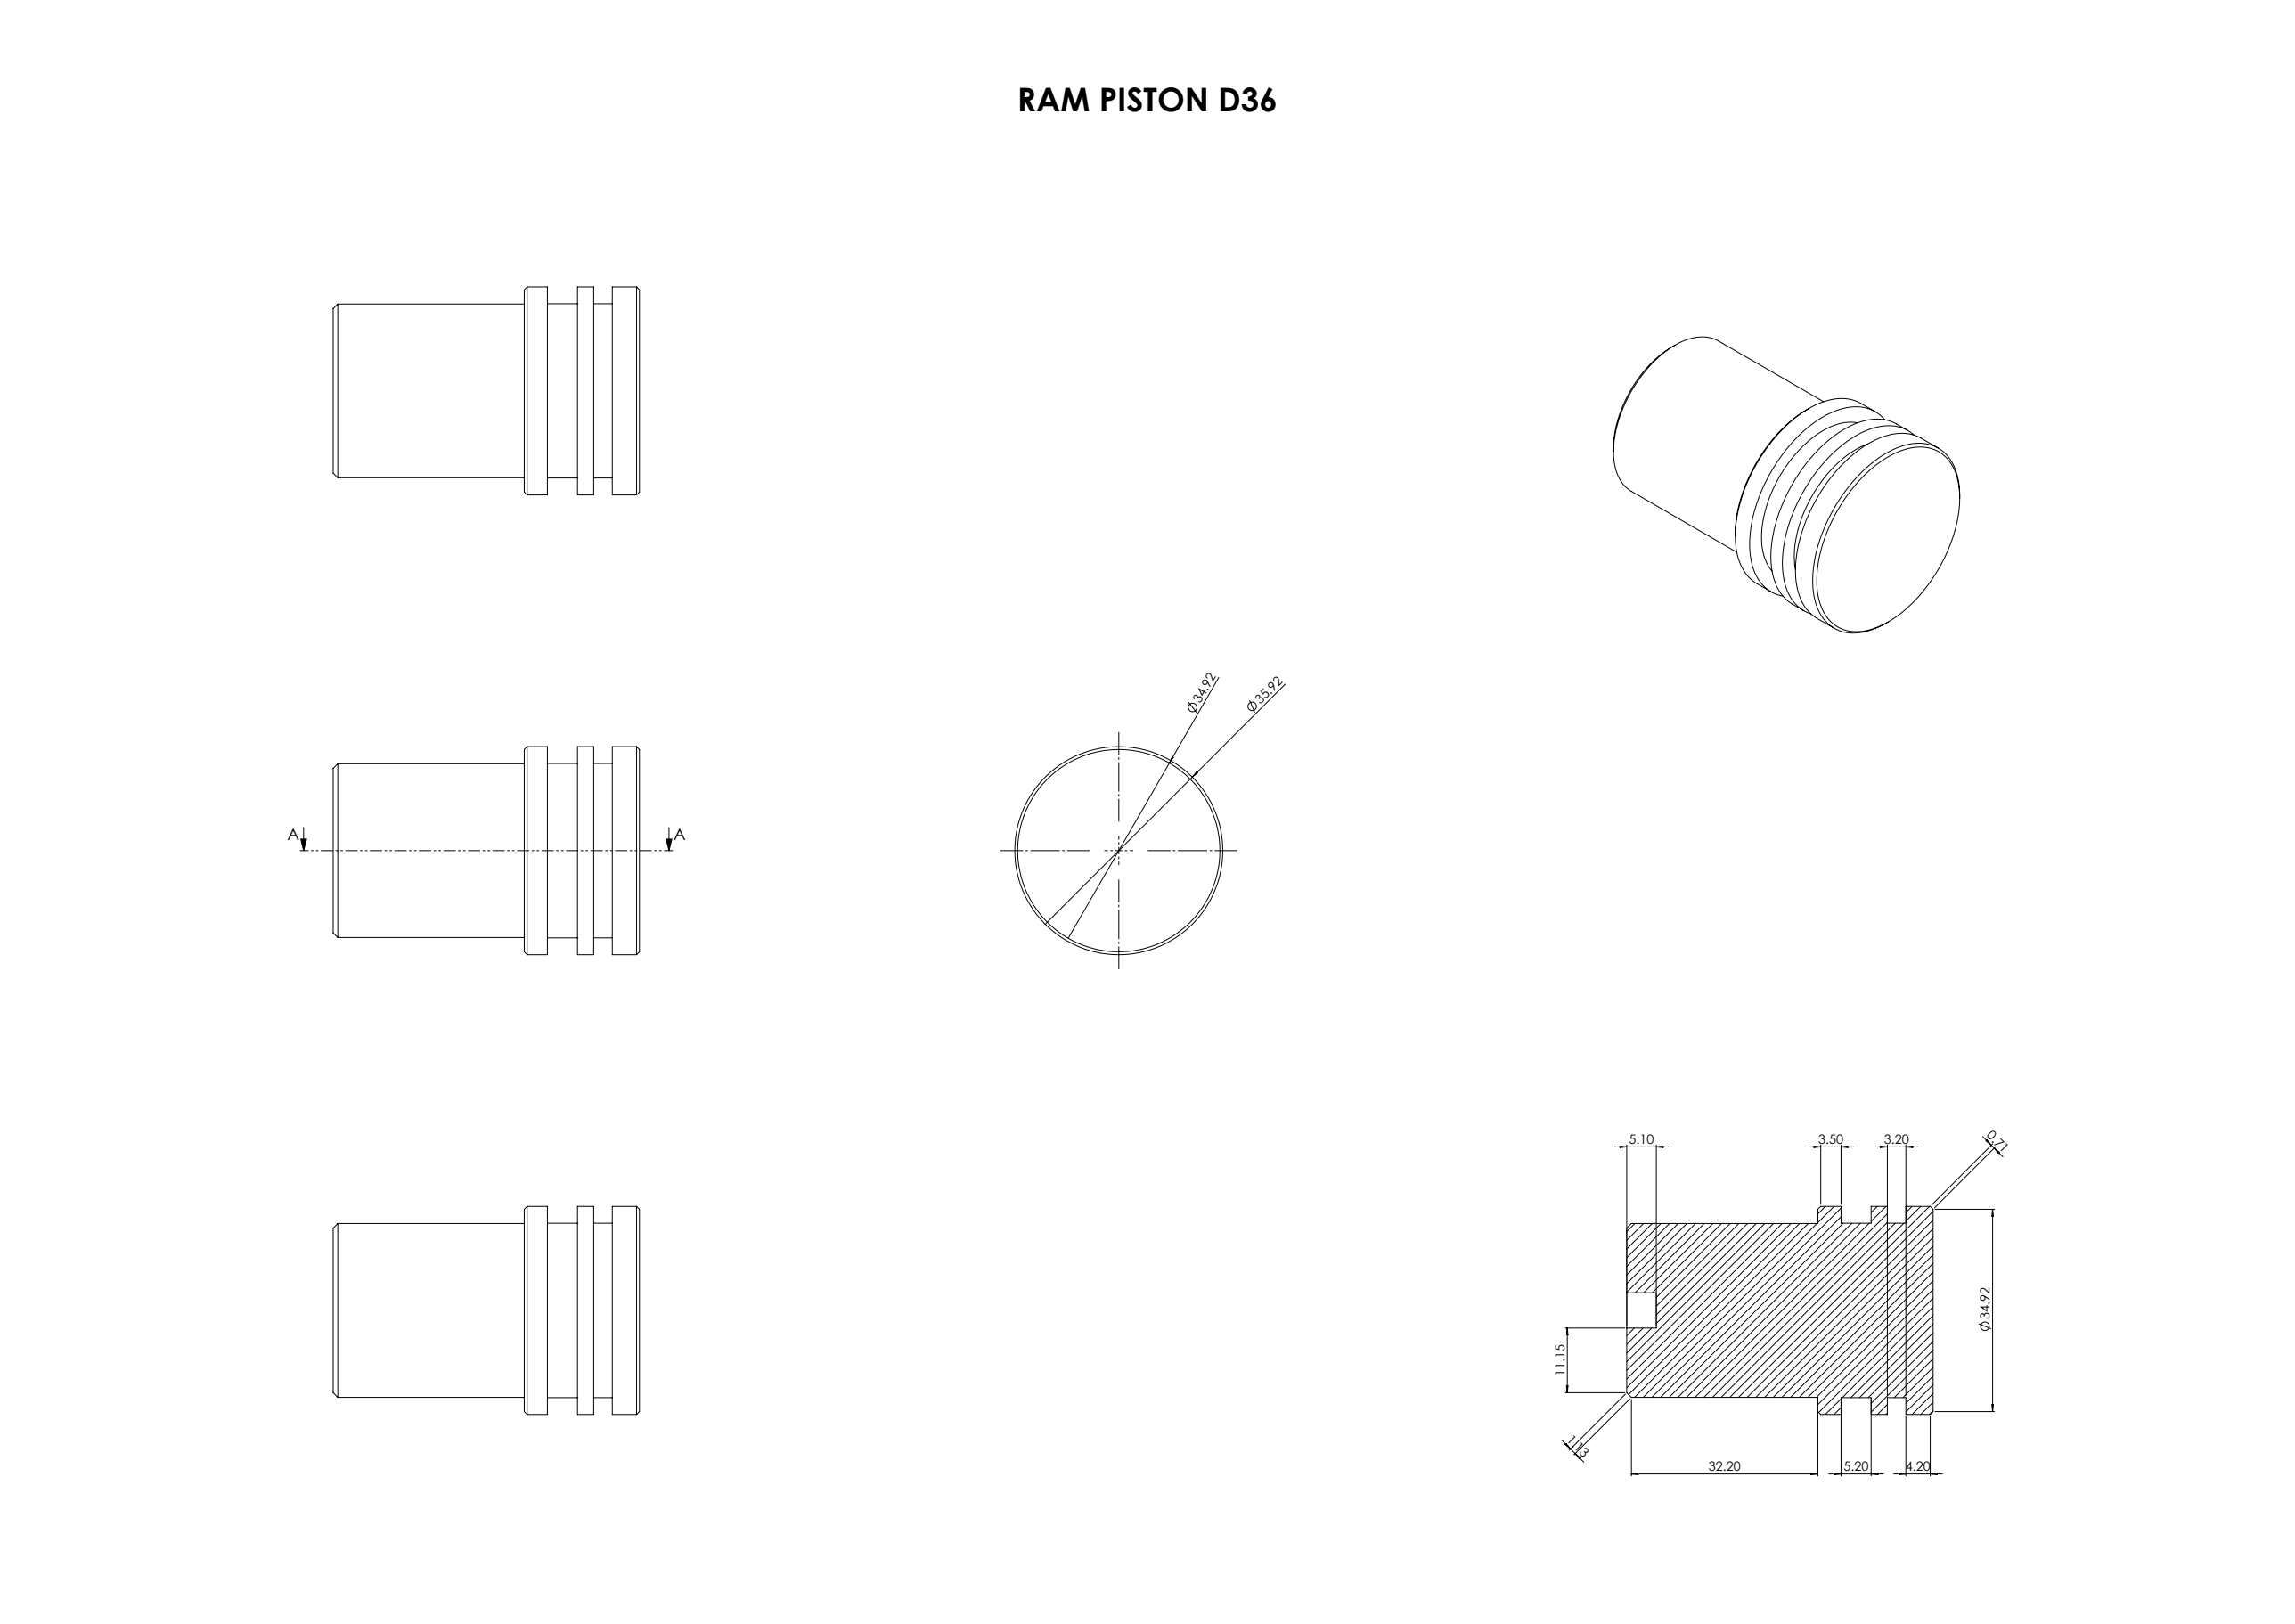
ISO-10303-21;
HEADER;
/* Generated by software containing ST-Developer
 * from STEP Tools, Inc. (www.steptools.com) 
 */

FILE_DESCRIPTION(
/* description */ (''),
/* implementation_level */ '2;1');

FILE_NAME(
/* name */ '03_Ram_Piston_D36.step',
/* time_stamp */ '2026-10-26T03:55:20-07:00',
/* author */ (''),
/* organization */ (''),
/* preprocessor_version */ 'ST-DEVELOPER v20.2',
/* originating_system */ 'Autodesk Translation Framework v15.15.0.0',
/* authorisation */ '');

FILE_SCHEMA (('AUTOMOTIVE_DESIGN { 1 0 10303 214 3 1 1 }'));
ENDSEC;

DATA;
#10=MECHANICAL_DESIGN_GEOMETRIC_PRESENTATION_REPRESENTATION('',(#177),#45236);
#137=SHAPE_REPRESENTATION_RELATIONSHIP('SRR','None',#45316,#157);
#157=ADVANCED_BREP_SHAPE_REPRESENTATION('',(#197),#45218);
#177=STYLED_ITEM('',(#45498),#197);
#197=MANIFOLD_SOLID_BREP('Body1',#16519);
#957=FACE_BOUND('',#3065,.T.);
#958=FACE_BOUND('',#3069,.T.);
#959=FACE_BOUND('',#3073,.T.);
#960=FACE_BOUND('',#3076,.T.);
#961=FACE_BOUND('',#3079,.T.);
#962=FACE_BOUND('',#3082,.T.);
#1122=PLANE('',#17115);
#1123=PLANE('',#17116);
#1124=PLANE('',#17122);
#1125=PLANE('',#17128);
#1126=PLANE('',#17132);
#1127=PLANE('',#17136);
#1128=PLANE('',#17140);
#1129=PLANE('',#17146);
#1674=CYLINDRICAL_SURFACE('',#17112,3.05);
#1675=CYLINDRICAL_SURFACE('',#17120,15.);
#1676=CYLINDRICAL_SURFACE('',#17126,17.96);
#1677=CYLINDRICAL_SURFACE('',#17130,15.05);
#1678=CYLINDRICAL_SURFACE('',#17134,17.96);
#1679=CYLINDRICAL_SURFACE('',#17138,15.05);
#1680=CYLINDRICAL_SURFACE('',#17142,17.96);
#2070=FACE_OUTER_BOUND('',#3062,.T.);
#2071=FACE_OUTER_BOUND('',#3063,.T.);
#2072=FACE_OUTER_BOUND('',#3064,.T.);
#2073=FACE_OUTER_BOUND('',#3066,.T.);
#2074=FACE_OUTER_BOUND('',#3067,.T.);
#2075=FACE_OUTER_BOUND('',#3068,.T.);
#2076=FACE_OUTER_BOUND('',#3070,.T.);
#2077=FACE_OUTER_BOUND('',#3071,.T.);
#2078=FACE_OUTER_BOUND('',#3072,.T.);
#2079=FACE_OUTER_BOUND('',#3074,.T.);
#2080=FACE_OUTER_BOUND('',#3075,.T.);
#2081=FACE_OUTER_BOUND('',#3077,.T.);
#2082=FACE_OUTER_BOUND('',#3078,.T.);
#2083=FACE_OUTER_BOUND('',#3080,.T.);
#2084=FACE_OUTER_BOUND('',#3081,.T.);
#2085=FACE_OUTER_BOUND('',#3083,.T.);
#2086=FACE_OUTER_BOUND('',#3084,.T.);
#2087=FACE_OUTER_BOUND('',#3085,.T.);
#3062=EDGE_LOOP('',(#12074,#12075,#12076,#12077));
#3063=EDGE_LOOP('',(#12078));
#3064=EDGE_LOOP('',(#12079));
#3065=EDGE_LOOP('',(#12080));
#3066=EDGE_LOOP('',(#12081,#12082,#12083,#12084));
#3067=EDGE_LOOP('',(#12085,#12086,#12087,#12088));
#3068=EDGE_LOOP('',(#12089));
#3069=EDGE_LOOP('',(#12090));
#3070=EDGE_LOOP('',(#12091,#12092,#12093,#12094));
#3071=EDGE_LOOP('',(#12095,#12096,#12097,#12098));
#3072=EDGE_LOOP('',(#12099));
#3073=EDGE_LOOP('',(#12100));
#3074=EDGE_LOOP('',(#12101,#12102,#12103,#12104));
#3075=EDGE_LOOP('',(#12105));
#3076=EDGE_LOOP('',(#12106));
#3077=EDGE_LOOP('',(#12107,#12108,#12109,#12110));
#3078=EDGE_LOOP('',(#12111));
#3079=EDGE_LOOP('',(#12112));
#3080=EDGE_LOOP('',(#12113,#12114,#12115,#12116));
#3081=EDGE_LOOP('',(#12117));
#3082=EDGE_LOOP('',(#12118));
#3083=EDGE_LOOP('',(#12119,#12120,#12121,#12122));
#3084=EDGE_LOOP('',(#12123,#12124,#12125,#12126));
#3085=EDGE_LOOP('',(#12127));
#4156=LINE('',#31337,#5467);
#4157=LINE('',#31346,#5468);
#4158=LINE('',#31350,#5469);
#4159=LINE('',#31357,#5470);
#4160=LINE('',#31361,#5471);
#4161=LINE('',#31368,#5472);
#4162=LINE('',#31375,#5473);
#4163=LINE('',#31382,#5474);
#4164=LINE('',#31389,#5475);
#4165=LINE('',#31393,#5476);
#5467=VECTOR('',#19105,3.05);
#5468=VECTOR('',#19118,14.6);
#5469=VECTOR('',#19123,15.);
#5470=VECTOR('',#19132,17.71);
#5471=VECTOR('',#19137,17.96);
#5472=VECTOR('',#19146,15.05);
#5473=VECTOR('',#19155,17.96);
#5474=VECTOR('',#19164,15.05);
#5475=VECTOR('',#19173,17.96);
#5476=VECTOR('',#19178,17.71);
#6644=CIRCLE('',#17113,3.05);
#6645=CIRCLE('',#17114,3.05);
#6646=CIRCLE('',#17117,14.2);
#6647=CIRCLE('',#17119,15.);
#6648=CIRCLE('',#17121,15.);
#6649=CIRCLE('',#17123,17.46);
#6650=CIRCLE('',#17125,17.96);
#6651=CIRCLE('',#17127,17.96);
#6652=CIRCLE('',#17129,15.05);
#6653=CIRCLE('',#17131,15.05);
#6654=CIRCLE('',#17133,17.96);
#6655=CIRCLE('',#17135,17.96);
#6656=CIRCLE('',#17137,15.05);
#6657=CIRCLE('',#17139,15.05);
#6658=CIRCLE('',#17141,17.96);
#6659=CIRCLE('',#17143,17.96);
#6660=CIRCLE('',#17145,17.46);
#7360=VERTEX_POINT('',#31334);
#7361=VERTEX_POINT('',#31336);
#7362=VERTEX_POINT('',#31341);
#7363=VERTEX_POINT('',#31344);
#7364=VERTEX_POINT('',#31348);
#7365=VERTEX_POINT('',#31352);
#7366=VERTEX_POINT('',#31355);
#7367=VERTEX_POINT('',#31359);
#7368=VERTEX_POINT('',#31363);
#7369=VERTEX_POINT('',#31366);
#7370=VERTEX_POINT('',#31370);
#7371=VERTEX_POINT('',#31373);
#7372=VERTEX_POINT('',#31377);
#7373=VERTEX_POINT('',#31380);
#7374=VERTEX_POINT('',#31384);
#7375=VERTEX_POINT('',#31387);
#7376=VERTEX_POINT('',#31391);
#9100=EDGE_CURVE('',#7360,#7360,#6644,.T.);
#9101=EDGE_CURVE('',#7360,#7361,#4156,.T.);
#9102=EDGE_CURVE('',#7361,#7361,#6645,.T.);
#9103=EDGE_CURVE('',#7362,#7362,#6646,.T.);
#9104=EDGE_CURVE('',#7363,#7363,#6647,.T.);
#9105=EDGE_CURVE('',#7363,#7362,#4157,.T.);
#9106=EDGE_CURVE('',#7364,#7364,#6648,.T.);
#9107=EDGE_CURVE('',#7364,#7363,#4158,.T.);
#9108=EDGE_CURVE('',#7365,#7365,#6649,.T.);
#9109=EDGE_CURVE('',#7366,#7366,#6650,.T.);
#9110=EDGE_CURVE('',#7366,#7365,#4159,.T.);
#9111=EDGE_CURVE('',#7367,#7367,#6651,.T.);
#9112=EDGE_CURVE('',#7367,#7366,#4160,.T.);
#9113=EDGE_CURVE('',#7368,#7368,#6652,.T.);
#9114=EDGE_CURVE('',#7369,#7369,#6653,.T.);
#9115=EDGE_CURVE('',#7369,#7368,#4161,.T.);
#9116=EDGE_CURVE('',#7370,#7370,#6654,.T.);
#9117=EDGE_CURVE('',#7371,#7371,#6655,.T.);
#9118=EDGE_CURVE('',#7371,#7370,#4162,.T.);
#9119=EDGE_CURVE('',#7372,#7372,#6656,.T.);
#9120=EDGE_CURVE('',#7373,#7373,#6657,.T.);
#9121=EDGE_CURVE('',#7373,#7372,#4163,.T.);
#9122=EDGE_CURVE('',#7374,#7374,#6658,.T.);
#9123=EDGE_CURVE('',#7375,#7375,#6659,.T.);
#9124=EDGE_CURVE('',#7375,#7374,#4164,.T.);
#9125=EDGE_CURVE('',#7376,#7376,#6660,.T.);
#9126=EDGE_CURVE('',#7376,#7375,#4165,.T.);
#12074=ORIENTED_EDGE('',*,*,#9100,.F.);
#12075=ORIENTED_EDGE('',*,*,#9101,.T.);
#12076=ORIENTED_EDGE('',*,*,#9102,.T.);
#12077=ORIENTED_EDGE('',*,*,#9101,.F.);
#12078=ORIENTED_EDGE('',*,*,#9102,.F.);
#12079=ORIENTED_EDGE('',*,*,#9103,.F.);
#12080=ORIENTED_EDGE('',*,*,#9100,.T.);
#12081=ORIENTED_EDGE('',*,*,#9104,.F.);
#12082=ORIENTED_EDGE('',*,*,#9105,.T.);
#12083=ORIENTED_EDGE('',*,*,#9103,.T.);
#12084=ORIENTED_EDGE('',*,*,#9105,.F.);
#12085=ORIENTED_EDGE('',*,*,#9106,.F.);
#12086=ORIENTED_EDGE('',*,*,#9107,.T.);
#12087=ORIENTED_EDGE('',*,*,#9104,.T.);
#12088=ORIENTED_EDGE('',*,*,#9107,.F.);
#12089=ORIENTED_EDGE('',*,*,#9108,.F.);
#12090=ORIENTED_EDGE('',*,*,#9106,.T.);
#12091=ORIENTED_EDGE('',*,*,#9109,.F.);
#12092=ORIENTED_EDGE('',*,*,#9110,.T.);
#12093=ORIENTED_EDGE('',*,*,#9108,.T.);
#12094=ORIENTED_EDGE('',*,*,#9110,.F.);
#12095=ORIENTED_EDGE('',*,*,#9111,.F.);
#12096=ORIENTED_EDGE('',*,*,#9112,.T.);
#12097=ORIENTED_EDGE('',*,*,#9109,.T.);
#12098=ORIENTED_EDGE('',*,*,#9112,.F.);
#12099=ORIENTED_EDGE('',*,*,#9111,.T.);
#12100=ORIENTED_EDGE('',*,*,#9113,.F.);
#12101=ORIENTED_EDGE('',*,*,#9114,.F.);
#12102=ORIENTED_EDGE('',*,*,#9115,.T.);
#12103=ORIENTED_EDGE('',*,*,#9113,.T.);
#12104=ORIENTED_EDGE('',*,*,#9115,.F.);
#12105=ORIENTED_EDGE('',*,*,#9116,.F.);
#12106=ORIENTED_EDGE('',*,*,#9114,.T.);
#12107=ORIENTED_EDGE('',*,*,#9117,.F.);
#12108=ORIENTED_EDGE('',*,*,#9118,.T.);
#12109=ORIENTED_EDGE('',*,*,#9116,.T.);
#12110=ORIENTED_EDGE('',*,*,#9118,.F.);
#12111=ORIENTED_EDGE('',*,*,#9117,.T.);
#12112=ORIENTED_EDGE('',*,*,#9119,.F.);
#12113=ORIENTED_EDGE('',*,*,#9120,.F.);
#12114=ORIENTED_EDGE('',*,*,#9121,.T.);
#12115=ORIENTED_EDGE('',*,*,#9119,.T.);
#12116=ORIENTED_EDGE('',*,*,#9121,.F.);
#12117=ORIENTED_EDGE('',*,*,#9122,.F.);
#12118=ORIENTED_EDGE('',*,*,#9120,.T.);
#12119=ORIENTED_EDGE('',*,*,#9123,.F.);
#12120=ORIENTED_EDGE('',*,*,#9124,.T.);
#12121=ORIENTED_EDGE('',*,*,#9122,.T.);
#12122=ORIENTED_EDGE('',*,*,#9124,.F.);
#12123=ORIENTED_EDGE('',*,*,#9125,.F.);
#12124=ORIENTED_EDGE('',*,*,#9126,.T.);
#12125=ORIENTED_EDGE('',*,*,#9123,.T.);
#12126=ORIENTED_EDGE('',*,*,#9126,.F.);
#12127=ORIENTED_EDGE('',*,*,#9125,.T.);
#15495=CONICAL_SURFACE('',#17118,14.6,0.785398163397454);
#15496=CONICAL_SURFACE('',#17124,17.71,0.785398163397442);
#15497=CONICAL_SURFACE('',#17144,17.71,0.785398163397459);
#15798=ADVANCED_FACE('',(#2070),#1674,.F.);
#15799=ADVANCED_FACE('',(#2071),#1122,.F.);
#15800=ADVANCED_FACE('',(#2072,#957),#1123,.T.);
#15801=ADVANCED_FACE('',(#2073),#15495,.T.);
#15802=ADVANCED_FACE('',(#2074),#1675,.T.);
#15803=ADVANCED_FACE('',(#2075,#958),#1124,.T.);
#15804=ADVANCED_FACE('',(#2076),#15496,.T.);
#15805=ADVANCED_FACE('',(#2077),#1676,.T.);
#15806=ADVANCED_FACE('',(#2078,#959),#1125,.T.);
#15807=ADVANCED_FACE('',(#2079),#1677,.T.);
#15808=ADVANCED_FACE('',(#2080,#960),#1126,.T.);
#15809=ADVANCED_FACE('',(#2081),#1678,.T.);
#15810=ADVANCED_FACE('',(#2082,#961),#1127,.T.);
#15811=ADVANCED_FACE('',(#2083),#1679,.T.);
#15812=ADVANCED_FACE('',(#2084,#962),#1128,.T.);
#15813=ADVANCED_FACE('',(#2085),#1680,.T.);
#15814=ADVANCED_FACE('',(#2086),#15497,.T.);
#15815=ADVANCED_FACE('',(#2087),#1129,.T.);
#16519=CLOSED_SHELL('',(#15798,#15799,#15800,#15801,#15802,#15803,#15804,
#15805,#15806,#15807,#15808,#15809,#15810,#15811,#15812,#15813,#15814,#15815));
#17111=AXIS2_PLACEMENT_3D('',#31332,#19099,#19100);
#17112=AXIS2_PLACEMENT_3D('',#31333,#19101,#19102);
#17113=AXIS2_PLACEMENT_3D('',#31335,#19103,#19104);
#17114=AXIS2_PLACEMENT_3D('',#31338,#19106,#19107);
#17115=AXIS2_PLACEMENT_3D('',#31339,#19108,#19109);
#17116=AXIS2_PLACEMENT_3D('',#31340,#19110,#19111);
#17117=AXIS2_PLACEMENT_3D('',#31342,#19112,#19113);
#17118=AXIS2_PLACEMENT_3D('',#31343,#19114,#19115);
#17119=AXIS2_PLACEMENT_3D('',#31345,#19116,#19117);
#17120=AXIS2_PLACEMENT_3D('',#31347,#19119,#19120);
#17121=AXIS2_PLACEMENT_3D('',#31349,#19121,#19122);
#17122=AXIS2_PLACEMENT_3D('',#31351,#19124,#19125);
#17123=AXIS2_PLACEMENT_3D('',#31353,#19126,#19127);
#17124=AXIS2_PLACEMENT_3D('',#31354,#19128,#19129);
#17125=AXIS2_PLACEMENT_3D('',#31356,#19130,#19131);
#17126=AXIS2_PLACEMENT_3D('',#31358,#19133,#19134);
#17127=AXIS2_PLACEMENT_3D('',#31360,#19135,#19136);
#17128=AXIS2_PLACEMENT_3D('',#31362,#19138,#19139);
#17129=AXIS2_PLACEMENT_3D('',#31364,#19140,#19141);
#17130=AXIS2_PLACEMENT_3D('',#31365,#19142,#19143);
#17131=AXIS2_PLACEMENT_3D('',#31367,#19144,#19145);
#17132=AXIS2_PLACEMENT_3D('',#31369,#19147,#19148);
#17133=AXIS2_PLACEMENT_3D('',#31371,#19149,#19150);
#17134=AXIS2_PLACEMENT_3D('',#31372,#19151,#19152);
#17135=AXIS2_PLACEMENT_3D('',#31374,#19153,#19154);
#17136=AXIS2_PLACEMENT_3D('',#31376,#19156,#19157);
#17137=AXIS2_PLACEMENT_3D('',#31378,#19158,#19159);
#17138=AXIS2_PLACEMENT_3D('',#31379,#19160,#19161);
#17139=AXIS2_PLACEMENT_3D('',#31381,#19162,#19163);
#17140=AXIS2_PLACEMENT_3D('',#31383,#19165,#19166);
#17141=AXIS2_PLACEMENT_3D('',#31385,#19167,#19168);
#17142=AXIS2_PLACEMENT_3D('',#31386,#19169,#19170);
#17143=AXIS2_PLACEMENT_3D('',#31388,#19171,#19172);
#17144=AXIS2_PLACEMENT_3D('',#31390,#19174,#19175);
#17145=AXIS2_PLACEMENT_3D('',#31392,#19176,#19177);
#17146=AXIS2_PLACEMENT_3D('',#31394,#19179,#19180);
#19099=DIRECTION('axis',(0.,0.,1.));
#19100=DIRECTION('refdir',(1.,0.,0.));
#19101=DIRECTION('center_axis',(1.,0.,0.));
#19102=DIRECTION('ref_axis',(0.,0.,-1.));
#19103=DIRECTION('center_axis',(1.,0.,0.));
#19104=DIRECTION('ref_axis',(0.,0.,-1.));
#19105=DIRECTION('',(1.,0.,0.));
#19106=DIRECTION('center_axis',(1.,0.,0.));
#19107=DIRECTION('ref_axis',(0.,0.,-1.));
#19108=DIRECTION('center_axis',(1.,0.,0.));
#19109=DIRECTION('ref_axis',(0.,0.,-1.));
#19110=DIRECTION('center_axis',(-1.,0.,0.));
#19111=DIRECTION('ref_axis',(0.,0.,1.));
#19112=DIRECTION('center_axis',(1.,0.,0.));
#19113=DIRECTION('ref_axis',(0.,0.,-1.));
#19114=DIRECTION('center_axis',(1.,0.,0.));
#19115=DIRECTION('ref_axis',(0.,1.,0.));
#19116=DIRECTION('center_axis',(1.,0.,0.));
#19117=DIRECTION('ref_axis',(0.,0.,-1.));
#19118=DIRECTION('',(-0.707106781186544,0.707106781186551,8.65956056235498E-17));
#19119=DIRECTION('center_axis',(1.,0.,0.));
#19120=DIRECTION('ref_axis',(0.,1.,0.));
#19121=DIRECTION('center_axis',(1.,0.,0.));
#19122=DIRECTION('ref_axis',(0.,0.,-1.));
#19123=DIRECTION('',(-1.,0.,0.));
#19124=DIRECTION('center_axis',(-1.,0.,0.));
#19125=DIRECTION('ref_axis',(0.,0.,1.));
#19126=DIRECTION('center_axis',(1.,0.,0.));
#19127=DIRECTION('ref_axis',(0.,0.,-1.));
#19128=DIRECTION('center_axis',(1.,0.,0.));
#19129=DIRECTION('ref_axis',(0.,1.,0.));
#19130=DIRECTION('center_axis',(1.,0.,0.));
#19131=DIRECTION('ref_axis',(0.,0.,-1.));
#19132=DIRECTION('',(-0.707106781186552,0.707106781186543,8.65956056235487E-17));
#19133=DIRECTION('center_axis',(1.,0.,0.));
#19134=DIRECTION('ref_axis',(0.,1.,0.));
#19135=DIRECTION('center_axis',(1.,0.,0.));
#19136=DIRECTION('ref_axis',(0.,0.,-1.));
#19137=DIRECTION('',(-1.,0.,0.));
#19138=DIRECTION('center_axis',(1.,0.,0.));
#19139=DIRECTION('ref_axis',(0.,0.,-1.));
#19140=DIRECTION('center_axis',(1.,0.,0.));
#19141=DIRECTION('ref_axis',(0.,0.,-1.));
#19142=DIRECTION('center_axis',(1.,0.,0.));
#19143=DIRECTION('ref_axis',(0.,1.,0.));
#19144=DIRECTION('center_axis',(1.,0.,0.));
#19145=DIRECTION('ref_axis',(0.,0.,-1.));
#19146=DIRECTION('',(-1.,0.,0.));
#19147=DIRECTION('center_axis',(-1.,0.,0.));
#19148=DIRECTION('ref_axis',(0.,0.,1.));
#19149=DIRECTION('center_axis',(1.,0.,0.));
#19150=DIRECTION('ref_axis',(0.,0.,-1.));
#19151=DIRECTION('center_axis',(1.,0.,0.));
#19152=DIRECTION('ref_axis',(0.,1.,0.));
#19153=DIRECTION('center_axis',(1.,0.,0.));
#19154=DIRECTION('ref_axis',(0.,0.,-1.));
#19155=DIRECTION('',(-1.,0.,0.));
#19156=DIRECTION('center_axis',(1.,0.,0.));
#19157=DIRECTION('ref_axis',(0.,0.,-1.));
#19158=DIRECTION('center_axis',(1.,0.,0.));
#19159=DIRECTION('ref_axis',(0.,0.,-1.));
#19160=DIRECTION('center_axis',(1.,0.,0.));
#19161=DIRECTION('ref_axis',(0.,1.,0.));
#19162=DIRECTION('center_axis',(1.,0.,0.));
#19163=DIRECTION('ref_axis',(0.,0.,-1.));
#19164=DIRECTION('',(-1.,0.,0.));
#19165=DIRECTION('center_axis',(-1.,0.,0.));
#19166=DIRECTION('ref_axis',(0.,0.,1.));
#19167=DIRECTION('center_axis',(1.,0.,0.));
#19168=DIRECTION('ref_axis',(0.,0.,-1.));
#19169=DIRECTION('center_axis',(1.,0.,0.));
#19170=DIRECTION('ref_axis',(0.,1.,0.));
#19171=DIRECTION('center_axis',(1.,0.,0.));
#19172=DIRECTION('ref_axis',(0.,0.,-1.));
#19173=DIRECTION('',(-1.,0.,0.));
#19174=DIRECTION('center_axis',(-1.,0.,0.));
#19175=DIRECTION('ref_axis',(0.,1.,0.));
#19176=DIRECTION('center_axis',(1.,0.,0.));
#19177=DIRECTION('ref_axis',(0.,0.,-1.));
#19178=DIRECTION('',(-0.70710678118654,-0.707106781186555,-8.65956056235503E-17));
#19179=DIRECTION('center_axis',(1.,0.,0.));
#19180=DIRECTION('ref_axis',(0.,0.,-1.));
#31332=CARTESIAN_POINT('',(0.,0.,0.));
#31333=CARTESIAN_POINT('Origin',(57.,0.,0.));
#31334=CARTESIAN_POINT('',(57.,-3.73517273739943E-16,3.05));
#31335=CARTESIAN_POINT('Origin',(57.,0.,0.));
#31336=CARTESIAN_POINT('',(62.1,-3.73517273739943E-16,3.05));
#31337=CARTESIAN_POINT('',(57.,-3.73517273739943E-16,3.05));
#31338=CARTESIAN_POINT('Origin',(62.1,0.,0.));
#31339=CARTESIAN_POINT('Origin',(62.1,0.,0.));
#31340=CARTESIAN_POINT('Origin',(57.,14.2,0.));
#31341=CARTESIAN_POINT('',(57.,-14.2,-1.73899845478924E-15));
#31342=CARTESIAN_POINT('Origin',(57.,0.,0.));
#31343=CARTESIAN_POINT('Origin',(57.4,0.,0.));
#31344=CARTESIAN_POINT('',(57.8,-15.,-1.83697019872103E-15));
#31345=CARTESIAN_POINT('Origin',(57.8,0.,0.));
#31346=CARTESIAN_POINT('',(57.4,-14.6,-1.78798432675514E-15));
#31347=CARTESIAN_POINT('Origin',(73.9,0.,0.));
#31348=CARTESIAN_POINT('',(90.,-15.,-1.83697019872103E-15));
#31349=CARTESIAN_POINT('Origin',(90.,0.,0.));
#31350=CARTESIAN_POINT('',(73.9,-15.,-1.83697019872103E-15));
#31351=CARTESIAN_POINT('Origin',(90.,17.46,0.));
#31352=CARTESIAN_POINT('',(90.,-17.46,-2.13823331131128E-15));
#31353=CARTESIAN_POINT('Origin',(90.,0.,0.));
#31354=CARTESIAN_POINT('Origin',(90.25,0.,0.));
#31355=CARTESIAN_POINT('',(90.5,-17.96,-2.19946565126865E-15));
#31356=CARTESIAN_POINT('Origin',(90.5,0.,0.));
#31357=CARTESIAN_POINT('',(90.25,-17.71,-2.16884948128996E-15));
#31358=CARTESIAN_POINT('Origin',(92.25,0.,0.));
#31359=CARTESIAN_POINT('',(94.,-17.96,-2.19946565126865E-15));
#31360=CARTESIAN_POINT('Origin',(94.,0.,0.));
#31361=CARTESIAN_POINT('',(92.25,-17.96,-2.19946565126865E-15));
#31362=CARTESIAN_POINT('Origin',(94.,15.05,0.));
#31363=CARTESIAN_POINT('',(94.,-15.05,-1.84309343271677E-15));
#31364=CARTESIAN_POINT('Origin',(94.,0.,0.));
#31365=CARTESIAN_POINT('Origin',(96.6,0.,0.));
#31366=CARTESIAN_POINT('',(99.2,-15.05,-1.84309343271677E-15));
#31367=CARTESIAN_POINT('Origin',(99.2,0.,0.));
#31368=CARTESIAN_POINT('',(96.6,-15.05,-1.84309343271677E-15));
#31369=CARTESIAN_POINT('Origin',(99.2,17.96,0.));
#31370=CARTESIAN_POINT('',(99.2,-17.96,-2.19946565126865E-15));
#31371=CARTESIAN_POINT('Origin',(99.2,0.,0.));
#31372=CARTESIAN_POINT('Origin',(100.6,0.,0.));
#31373=CARTESIAN_POINT('',(102.,-17.96,-2.19946565126865E-15));
#31374=CARTESIAN_POINT('Origin',(102.,0.,0.));
#31375=CARTESIAN_POINT('',(100.6,-17.96,-2.19946565126865E-15));
#31376=CARTESIAN_POINT('Origin',(102.,15.05,0.));
#31377=CARTESIAN_POINT('',(102.,-15.05,-1.84309343271677E-15));
#31378=CARTESIAN_POINT('Origin',(102.,0.,0.));
#31379=CARTESIAN_POINT('Origin',(103.6,0.,0.));
#31380=CARTESIAN_POINT('',(105.2,-15.05,-1.84309343271677E-15));
#31381=CARTESIAN_POINT('Origin',(105.2,0.,0.));
#31382=CARTESIAN_POINT('',(103.6,-15.05,-1.84309343271677E-15));
#31383=CARTESIAN_POINT('Origin',(105.2,17.96,0.));
#31384=CARTESIAN_POINT('',(105.2,-17.96,-2.19946565126865E-15));
#31385=CARTESIAN_POINT('Origin',(105.2,0.,0.));
#31386=CARTESIAN_POINT('Origin',(107.3,0.,0.));
#31387=CARTESIAN_POINT('',(109.4,-17.96,-2.19946565126865E-15));
#31388=CARTESIAN_POINT('Origin',(109.4,0.,0.));
#31389=CARTESIAN_POINT('',(107.3,-17.96,-2.19946565126865E-15));
#31390=CARTESIAN_POINT('Origin',(109.65,0.,0.));
#31391=CARTESIAN_POINT('',(109.9,-17.46,-2.13823331131128E-15));
#31392=CARTESIAN_POINT('Origin',(109.9,0.,0.));
#31393=CARTESIAN_POINT('',(109.65,-17.71,-2.16884948128996E-15));
#31394=CARTESIAN_POINT('Origin',(109.9,0.,0.));
#45196=UNCERTAINTY_MEASURE_WITH_UNIT(LENGTH_MEASURE(0.01),#45237,
'DISTANCE_ACCURACY_VALUE',
'Maximum model space distance between geometric entities at asserted c
onnectivities');
#45214=UNCERTAINTY_MEASURE_WITH_UNIT(LENGTH_MEASURE(0.01),#45237,
'DISTANCE_ACCURACY_VALUE',
'Maximum model space distance between geometric entities at asserted c
onnectivities');
#45218=(
GEOMETRIC_REPRESENTATION_CONTEXT(3)
GLOBAL_UNCERTAINTY_ASSIGNED_CONTEXT((#45196))
GLOBAL_UNIT_ASSIGNED_CONTEXT((#45237,#45239,#45240))
REPRESENTATION_CONTEXT('','3D')
);
#45236=(
GEOMETRIC_REPRESENTATION_CONTEXT(3)
GLOBAL_UNCERTAINTY_ASSIGNED_CONTEXT((#45214))
GLOBAL_UNIT_ASSIGNED_CONTEXT((#45237,#45239,#45240))
REPRESENTATION_CONTEXT('','3D')
);
#45237=(
LENGTH_UNIT()
NAMED_UNIT(*)
SI_UNIT(.MILLI.,.METRE.)
);
#45239=(
NAMED_UNIT(*)
PLANE_ANGLE_UNIT()
SI_UNIT($,.RADIAN.)
);
#45240=(
NAMED_UNIT(*)
SI_UNIT($,.STERADIAN.)
SOLID_ANGLE_UNIT()
);
#45244=SHAPE_DEFINITION_REPRESENTATION(#45265,#45316);
#45265=PRODUCT_DEFINITION_SHAPE('',$,#45338);
#45316=SHAPE_REPRESENTATION('',(#17111),#45218);
#45334=PRODUCT_DEFINITION_CONTEXT('part definition',#45399,'design');
#45338=PRODUCT_DEFINITION('2026-10-25-23-38-15-275','03_Ram_Piston_D36',
#45359,#45334);
#45359=PRODUCT_DEFINITION_FORMATION('',$,#45404);
#45399=APPLICATION_CONTEXT(
'Core Data for Automotive Mechanical Design Process');
#45400=PRODUCT_CONTEXT('part definition',#45399,'mechanical');
#45404=PRODUCT('2026-10-25-23-38-15-275','03_Ram_Piston_D36',$,(#45400));
#45492=COLOUR_RGB('Off White',0.89,0.88,0.83);
#45493=FILL_AREA_STYLE_COLOUR('',#45492);
#45494=FILL_AREA_STYLE('',(#45493));
#45495=SURFACE_STYLE_FILL_AREA(#45494);
#45496=SURFACE_SIDE_STYLE('',(#45495));
#45497=SURFACE_STYLE_USAGE(.BOTH.,#45496);
#45498=PRESENTATION_STYLE_ASSIGNMENT((#45497));
ENDSEC;
END-ISO-10303-21;
